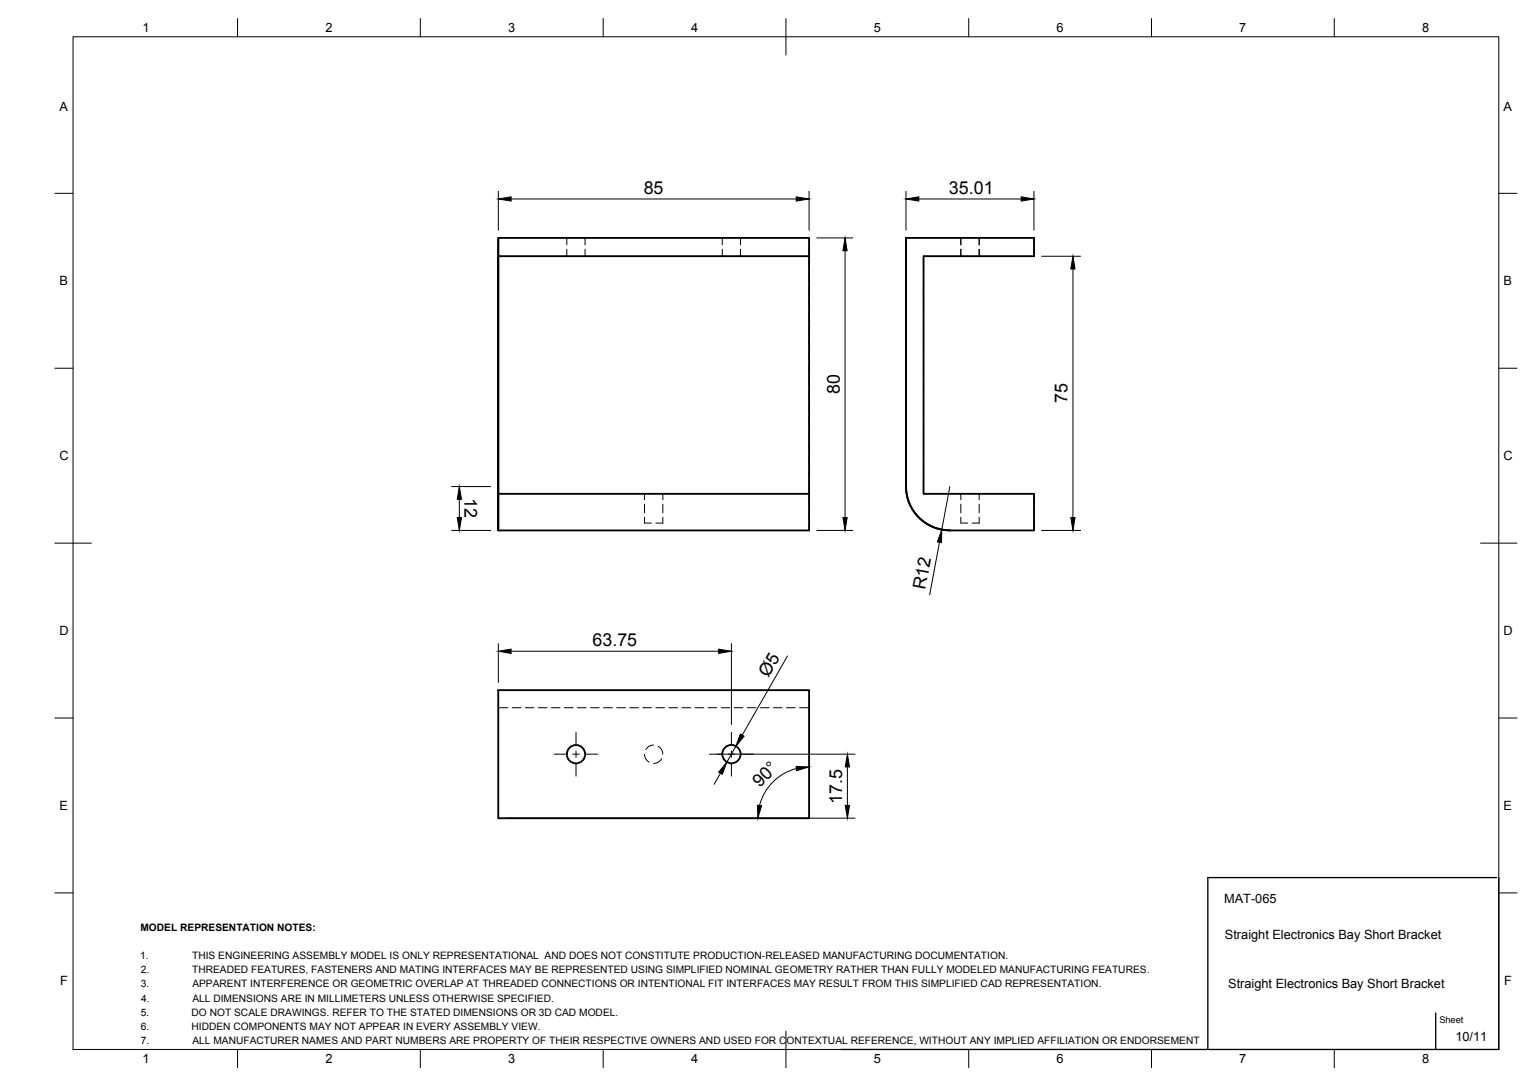
ISO-10303-21;
HEADER;
/* Generated by software containing ST-Developer
 * from STEP Tools, Inc. (www.steptools.com) 
 */

FILE_DESCRIPTION(
/* description */ (
'CAx-IF Rec.Pracs.---Representation and Presentation of Product Manufa
cturing Information (PMI)---4.0---2014-10-13'),
/* implementation_level */ '2;1');

FILE_NAME(
/* name */ 'Straight Electronics Bay Short Bracket.step',
/* time_stamp */ '2026-11-15T23:28:27-08:00',
/* author */ (''),
/* organization */ (''),
/* preprocessor_version */ 'ST-DEVELOPER v20.2',
/* originating_system */ 'Autodesk Translation Framework v15.17.0.0',
/* authorisation */ '');

FILE_SCHEMA (('AUTOMOTIVE_DESIGN { 1 0 10303 214 3 1 1 }'));
ENDSEC;

DATA;
#10=MECHANICAL_DESIGN_GEOMETRIC_PRESENTATION_REPRESENTATION('',(#191),#7756);
#173=SHAPE_REPRESENTATION_RELATIONSHIP('SRR','None',#7821,#182);
#182=ADVANCED_BREP_SHAPE_REPRESENTATION('',(#200),#7749);
#191=STYLED_ITEM('',(#7875),#200);
#200=MANIFOLD_SOLID_BREP('Body1',#4628);
#212=CYLINDRICAL_SURFACE('',#4780,0.0025);
#213=CYLINDRICAL_SURFACE('',#4783,0.0025);
#214=CYLINDRICAL_SURFACE('',#4793,0.012);
#215=CYLINDRICAL_SURFACE('',#4794,0.0025);
#274=CIRCLE('',#4775,0.012);
#275=CIRCLE('',#4778,0.012);
#276=CIRCLE('',#4781,0.0025);
#277=CIRCLE('',#4782,0.0025);
#278=CIRCLE('',#4784,0.0025);
#279=CIRCLE('',#4785,0.0025);
#280=CIRCLE('',#4790,0.0025);
#281=CIRCLE('',#4795,0.0025);
#392=FACE_BOUND('',#731,.T.);
#393=FACE_BOUND('',#732,.T.);
#394=FACE_BOUND('',#734,.T.);
#395=FACE_BOUND('',#735,.T.);
#396=FACE_BOUND('',#738,.T.);
#477=FACE_OUTER_BOUND('',#724,.T.);
#478=FACE_OUTER_BOUND('',#725,.T.);
#479=FACE_OUTER_BOUND('',#726,.T.);
#480=FACE_OUTER_BOUND('',#727,.T.);
#481=FACE_OUTER_BOUND('',#728,.T.);
#482=FACE_OUTER_BOUND('',#729,.T.);
#483=FACE_OUTER_BOUND('',#730,.T.);
#484=FACE_OUTER_BOUND('',#733,.T.);
#485=FACE_OUTER_BOUND('',#736,.T.);
#486=FACE_OUTER_BOUND('',#737,.T.);
#487=FACE_OUTER_BOUND('',#739,.T.);
#488=FACE_OUTER_BOUND('',#740,.T.);
#489=FACE_OUTER_BOUND('',#741,.T.);
#490=FACE_OUTER_BOUND('',#742,.T.);
#491=FACE_OUTER_BOUND('',#743,.T.);
#724=EDGE_LOOP('',(#3119,#3120,#3121,#3122,#3123,#3124,#3125,#3126,#3127));
#725=EDGE_LOOP('',(#3128,#3129,#3130,#3131));
#726=EDGE_LOOP('',(#3132,#3133,#3134,#3135,#3136,#3137,#3138,#3139,#3140));
#727=EDGE_LOOP('',(#3141,#3142,#3143,#3144));
#728=EDGE_LOOP('',(#3145,#3146,#3147,#3148));
#729=EDGE_LOOP('',(#3149,#3150,#3151,#3152));
#730=EDGE_LOOP('',(#3153,#3154,#3155,#3156));
#731=EDGE_LOOP('',(#3157));
#732=EDGE_LOOP('',(#3158));
#733=EDGE_LOOP('',(#3159,#3160,#3161,#3162));
#734=EDGE_LOOP('',(#3163));
#735=EDGE_LOOP('',(#3164));
#736=EDGE_LOOP('',(#3165,#3166,#3167,#3168));
#737=EDGE_LOOP('',(#3169,#3170,#3171,#3172));
#738=EDGE_LOOP('',(#3173));
#739=EDGE_LOOP('',(#3174,#3175,#3176,#3177));
#740=EDGE_LOOP('',(#3178,#3179,#3180,#3181));
#741=EDGE_LOOP('',(#3182,#3183,#3184,#3185));
#742=EDGE_LOOP('',(#3186,#3187,#3188,#3189));
#743=EDGE_LOOP('',(#3190));
#1045=LINE('',#6556,#1538);
#1046=LINE('',#6560,#1539);
#1047=LINE('',#6562,#1540);
#1048=LINE('',#6564,#1541);
#1049=LINE('',#6566,#1542);
#1050=LINE('',#6568,#1543);
#1051=LINE('',#6570,#1544);
#1052=LINE('',#6571,#1545);
#1053=LINE('',#6574,#1546);
#1054=LINE('',#6576,#1547);
#1055=LINE('',#6577,#1548);
#1056=LINE('',#6581,#1549);
#1057=LINE('',#6585,#1550);
#1058=LINE('',#6587,#1551);
#1059=LINE('',#6589,#1552);
#1060=LINE('',#6591,#1553);
#1061=LINE('',#6592,#1554);
#1062=LINE('',#6593,#1555);
#1063=LINE('',#6595,#1556);
#1064=LINE('',#6596,#1557);
#1065=LINE('',#6601,#1558);
#1066=LINE('',#6607,#1559);
#1067=LINE('',#6610,#1560);
#1068=LINE('',#6613,#1561);
#1069=LINE('',#6615,#1562);
#1070=LINE('',#6619,#1563);
#1071=LINE('',#6621,#1564);
#1072=LINE('',#6626,#1565);
#1538=VECTOR('',#5265,1.);
#1539=VECTOR('',#5268,1.);
#1540=VECTOR('',#5269,1.);
#1541=VECTOR('',#5270,1.);
#1542=VECTOR('',#5271,1.);
#1543=VECTOR('',#5272,1.);
#1544=VECTOR('',#5273,1.);
#1545=VECTOR('',#5274,1.);
#1546=VECTOR('',#5277,1.);
#1547=VECTOR('',#5278,1.);
#1548=VECTOR('',#5279,1.);
#1549=VECTOR('',#5282,1.);
#1550=VECTOR('',#5285,1.);
#1551=VECTOR('',#5286,1.);
#1552=VECTOR('',#5287,1.);
#1553=VECTOR('',#5288,1.);
#1554=VECTOR('',#5289,1.);
#1555=VECTOR('',#5290,1.);
#1556=VECTOR('',#5293,1.);
#1557=VECTOR('',#5294,1.);
#1558=VECTOR('',#5299,0.0025);
#1559=VECTOR('',#5306,0.0025);
#1560=VECTOR('',#5311,1.);
#1561=VECTOR('',#5316,1.);
#1562=VECTOR('',#5319,1.);
#1563=VECTOR('',#5324,1.);
#1564=VECTOR('',#5327,1.);
#1565=VECTOR('',#5334,0.0025);
#2020=VERTEX_POINT('',#6554);
#2021=VERTEX_POINT('',#6555);
#2022=VERTEX_POINT('',#6557);
#2023=VERTEX_POINT('',#6559);
#2024=VERTEX_POINT('',#6561);
#2025=VERTEX_POINT('',#6563);
#2026=VERTEX_POINT('',#6565);
#2027=VERTEX_POINT('',#6567);
#2028=VERTEX_POINT('',#6569);
#2029=VERTEX_POINT('',#6573);
#2030=VERTEX_POINT('',#6575);
#2031=VERTEX_POINT('',#6579);
#2032=VERTEX_POINT('',#6580);
#2033=VERTEX_POINT('',#6582);
#2034=VERTEX_POINT('',#6584);
#2035=VERTEX_POINT('',#6586);
#2036=VERTEX_POINT('',#6588);
#2037=VERTEX_POINT('',#6590);
#2038=VERTEX_POINT('',#6598);
#2039=VERTEX_POINT('',#6600);
#2040=VERTEX_POINT('',#6604);
#2041=VERTEX_POINT('',#6606);
#2042=VERTEX_POINT('',#6616);
#2043=VERTEX_POINT('',#6624);
#2443=EDGE_CURVE('',#2020,#2021,#1045,.T.);
#2444=EDGE_CURVE('',#2021,#2022,#274,.T.);
#2445=EDGE_CURVE('',#2022,#2023,#1046,.T.);
#2446=EDGE_CURVE('',#2024,#2023,#1047,.T.);
#2447=EDGE_CURVE('',#2025,#2024,#1048,.T.);
#2448=EDGE_CURVE('',#2025,#2026,#1049,.T.);
#2449=EDGE_CURVE('',#2027,#2026,#1050,.T.);
#2450=EDGE_CURVE('',#2028,#2027,#1051,.T.);
#2451=EDGE_CURVE('',#2020,#2028,#1052,.T.);
#2452=EDGE_CURVE('',#2024,#2029,#1053,.T.);
#2453=EDGE_CURVE('',#2030,#2029,#1054,.T.);
#2454=EDGE_CURVE('',#2025,#2030,#1055,.T.);
#2455=EDGE_CURVE('',#2031,#2032,#1056,.T.);
#2456=EDGE_CURVE('',#2031,#2033,#275,.F.);
#2457=EDGE_CURVE('',#2034,#2033,#1057,.T.);
#2458=EDGE_CURVE('',#2034,#2035,#1058,.T.);
#2459=EDGE_CURVE('',#2035,#2036,#1059,.T.);
#2460=EDGE_CURVE('',#2036,#2037,#1060,.T.);
#2461=EDGE_CURVE('',#2030,#2037,#1061,.T.);
#2462=EDGE_CURVE('',#2029,#2032,#1062,.T.);
#2463=EDGE_CURVE('',#2022,#2031,#1063,.T.);
#2464=EDGE_CURVE('',#2023,#2032,#1064,.T.);
#2465=EDGE_CURVE('',#2038,#2038,#276,.T.);
#2466=EDGE_CURVE('',#2038,#2039,#1065,.T.);
#2467=EDGE_CURVE('',#2039,#2039,#277,.T.);
#2468=EDGE_CURVE('',#2040,#2040,#278,.T.);
#2469=EDGE_CURVE('',#2040,#2041,#1066,.T.);
#2470=EDGE_CURVE('',#2041,#2041,#279,.T.);
#2471=EDGE_CURVE('',#2026,#2037,#1067,.T.);
#2472=EDGE_CURVE('',#2027,#2036,#1068,.T.);
#2473=EDGE_CURVE('',#2028,#2035,#1069,.T.);
#2474=EDGE_CURVE('',#2042,#2042,#280,.T.);
#2475=EDGE_CURVE('',#2020,#2034,#1070,.T.);
#2476=EDGE_CURVE('',#2033,#2021,#1071,.F.);
#2477=EDGE_CURVE('',#2043,#2043,#281,.T.);
#2478=EDGE_CURVE('',#2043,#2042,#1072,.T.);
#3119=ORIENTED_EDGE('',*,*,#2443,.T.);
#3120=ORIENTED_EDGE('',*,*,#2444,.T.);
#3121=ORIENTED_EDGE('',*,*,#2445,.T.);
#3122=ORIENTED_EDGE('',*,*,#2446,.F.);
#3123=ORIENTED_EDGE('',*,*,#2447,.F.);
#3124=ORIENTED_EDGE('',*,*,#2448,.T.);
#3125=ORIENTED_EDGE('',*,*,#2449,.F.);
#3126=ORIENTED_EDGE('',*,*,#2450,.F.);
#3127=ORIENTED_EDGE('',*,*,#2451,.F.);
#3128=ORIENTED_EDGE('',*,*,#2452,.T.);
#3129=ORIENTED_EDGE('',*,*,#2453,.F.);
#3130=ORIENTED_EDGE('',*,*,#2454,.F.);
#3131=ORIENTED_EDGE('',*,*,#2447,.T.);
#3132=ORIENTED_EDGE('',*,*,#2455,.F.);
#3133=ORIENTED_EDGE('',*,*,#2456,.T.);
#3134=ORIENTED_EDGE('',*,*,#2457,.F.);
#3135=ORIENTED_EDGE('',*,*,#2458,.T.);
#3136=ORIENTED_EDGE('',*,*,#2459,.T.);
#3137=ORIENTED_EDGE('',*,*,#2460,.T.);
#3138=ORIENTED_EDGE('',*,*,#2461,.F.);
#3139=ORIENTED_EDGE('',*,*,#2453,.T.);
#3140=ORIENTED_EDGE('',*,*,#2462,.T.);
#3141=ORIENTED_EDGE('',*,*,#2445,.F.);
#3142=ORIENTED_EDGE('',*,*,#2463,.T.);
#3143=ORIENTED_EDGE('',*,*,#2455,.T.);
#3144=ORIENTED_EDGE('',*,*,#2464,.F.);
#3145=ORIENTED_EDGE('',*,*,#2465,.F.);
#3146=ORIENTED_EDGE('',*,*,#2466,.T.);
#3147=ORIENTED_EDGE('',*,*,#2467,.T.);
#3148=ORIENTED_EDGE('',*,*,#2466,.F.);
#3149=ORIENTED_EDGE('',*,*,#2468,.F.);
#3150=ORIENTED_EDGE('',*,*,#2469,.T.);
#3151=ORIENTED_EDGE('',*,*,#2470,.T.);
#3152=ORIENTED_EDGE('',*,*,#2469,.F.);
#3153=ORIENTED_EDGE('',*,*,#2471,.F.);
#3154=ORIENTED_EDGE('',*,*,#2448,.F.);
#3155=ORIENTED_EDGE('',*,*,#2454,.T.);
#3156=ORIENTED_EDGE('',*,*,#2461,.T.);
#3157=ORIENTED_EDGE('',*,*,#2465,.T.);
#3158=ORIENTED_EDGE('',*,*,#2468,.T.);
#3159=ORIENTED_EDGE('',*,*,#2446,.T.);
#3160=ORIENTED_EDGE('',*,*,#2464,.T.);
#3161=ORIENTED_EDGE('',*,*,#2462,.F.);
#3162=ORIENTED_EDGE('',*,*,#2452,.F.);
#3163=ORIENTED_EDGE('',*,*,#2470,.F.);
#3164=ORIENTED_EDGE('',*,*,#2467,.F.);
#3165=ORIENTED_EDGE('',*,*,#2471,.T.);
#3166=ORIENTED_EDGE('',*,*,#2460,.F.);
#3167=ORIENTED_EDGE('',*,*,#2472,.F.);
#3168=ORIENTED_EDGE('',*,*,#2449,.T.);
#3169=ORIENTED_EDGE('',*,*,#2450,.T.);
#3170=ORIENTED_EDGE('',*,*,#2472,.T.);
#3171=ORIENTED_EDGE('',*,*,#2459,.F.);
#3172=ORIENTED_EDGE('',*,*,#2473,.F.);
#3173=ORIENTED_EDGE('',*,*,#2474,.F.);
#3174=ORIENTED_EDGE('',*,*,#2473,.T.);
#3175=ORIENTED_EDGE('',*,*,#2458,.F.);
#3176=ORIENTED_EDGE('',*,*,#2475,.F.);
#3177=ORIENTED_EDGE('',*,*,#2451,.T.);
#3178=ORIENTED_EDGE('',*,*,#2457,.T.);
#3179=ORIENTED_EDGE('',*,*,#2476,.T.);
#3180=ORIENTED_EDGE('',*,*,#2443,.F.);
#3181=ORIENTED_EDGE('',*,*,#2475,.T.);
#3182=ORIENTED_EDGE('',*,*,#2444,.F.);
#3183=ORIENTED_EDGE('',*,*,#2476,.F.);
#3184=ORIENTED_EDGE('',*,*,#2456,.F.);
#3185=ORIENTED_EDGE('',*,*,#2463,.F.);
#3186=ORIENTED_EDGE('',*,*,#2477,.F.);
#3187=ORIENTED_EDGE('',*,*,#2478,.T.);
#3188=ORIENTED_EDGE('',*,*,#2474,.T.);
#3189=ORIENTED_EDGE('',*,*,#2478,.F.);
#3190=ORIENTED_EDGE('',*,*,#2477,.T.);
#4239=PLANE('',#4774);
#4240=PLANE('',#4776);
#4241=PLANE('',#4777);
#4242=PLANE('',#4779);
#4243=PLANE('',#4786);
#4244=PLANE('',#4787);
#4245=PLANE('',#4788);
#4246=PLANE('',#4789);
#4247=PLANE('',#4791);
#4248=PLANE('',#4792);
#4249=PLANE('',#4796);
#4418=ADVANCED_FACE('',(#477),#4239,.T.);
#4419=ADVANCED_FACE('',(#478),#4240,.F.);
#4420=ADVANCED_FACE('',(#479),#4241,.F.);
#4421=ADVANCED_FACE('',(#480),#4242,.T.);
#4422=ADVANCED_FACE('',(#481),#212,.F.);
#4423=ADVANCED_FACE('',(#482),#213,.F.);
#4424=ADVANCED_FACE('',(#483,#392,#393),#4243,.T.);
#4425=ADVANCED_FACE('',(#484,#394,#395),#4244,.F.);
#4426=ADVANCED_FACE('',(#485),#4245,.F.);
#4427=ADVANCED_FACE('',(#486,#396),#4246,.F.);
#4428=ADVANCED_FACE('',(#487),#4247,.F.);
#4429=ADVANCED_FACE('',(#488),#4248,.T.);
#4430=ADVANCED_FACE('',(#489),#214,.T.);
#4431=ADVANCED_FACE('',(#490),#215,.F.);
#4432=ADVANCED_FACE('',(#491),#4249,.T.);
#4628=CLOSED_SHELL('',(#4418,#4419,#4420,#4421,#4422,#4423,#4424,#4425,
#4426,#4427,#4428,#4429,#4430,#4431,#4432));
#4773=AXIS2_PLACEMENT_3D('',#6552,#5261,#5262);
#4774=AXIS2_PLACEMENT_3D('',#6553,#5263,#5264);
#4775=AXIS2_PLACEMENT_3D('',#6558,#5266,#5267);
#4776=AXIS2_PLACEMENT_3D('',#6572,#5275,#5276);
#4777=AXIS2_PLACEMENT_3D('',#6578,#5280,#5281);
#4778=AXIS2_PLACEMENT_3D('',#6583,#5283,#5284);
#4779=AXIS2_PLACEMENT_3D('',#6594,#5291,#5292);
#4780=AXIS2_PLACEMENT_3D('',#6597,#5295,#5296);
#4781=AXIS2_PLACEMENT_3D('',#6599,#5297,#5298);
#4782=AXIS2_PLACEMENT_3D('',#6602,#5300,#5301);
#4783=AXIS2_PLACEMENT_3D('',#6603,#5302,#5303);
#4784=AXIS2_PLACEMENT_3D('',#6605,#5304,#5305);
#4785=AXIS2_PLACEMENT_3D('',#6608,#5307,#5308);
#4786=AXIS2_PLACEMENT_3D('',#6609,#5309,#5310);
#4787=AXIS2_PLACEMENT_3D('',#6611,#5312,#5313);
#4788=AXIS2_PLACEMENT_3D('',#6612,#5314,#5315);
#4789=AXIS2_PLACEMENT_3D('',#6614,#5317,#5318);
#4790=AXIS2_PLACEMENT_3D('',#6617,#5320,#5321);
#4791=AXIS2_PLACEMENT_3D('',#6618,#5322,#5323);
#4792=AXIS2_PLACEMENT_3D('',#6620,#5325,#5326);
#4793=AXIS2_PLACEMENT_3D('',#6622,#5328,#5329);
#4794=AXIS2_PLACEMENT_3D('',#6623,#5330,#5331);
#4795=AXIS2_PLACEMENT_3D('',#6625,#5332,#5333);
#4796=AXIS2_PLACEMENT_3D('',#6627,#5335,#5336);
#5261=DIRECTION('axis',(0.,0.,1.));
#5262=DIRECTION('refdir',(1.,0.,0.));
#5263=DIRECTION('center_axis',(-1.,0.,0.));
#5264=DIRECTION('ref_axis',(0.,0.,1.));
#5265=DIRECTION('',(0.,-1.,0.));
#5266=DIRECTION('center_axis',(-1.,0.,0.));
#5267=DIRECTION('ref_axis',(0.,0.,1.));
#5268=DIRECTION('',(0.,0.,1.));
#5269=DIRECTION('',(0.,-1.,0.));
#5270=DIRECTION('',(0.,0.,1.));
#5271=DIRECTION('',(0.,-1.,0.));
#5272=DIRECTION('',(0.,0.,1.));
#5273=DIRECTION('',(0.,-1.,0.));
#5274=DIRECTION('',(0.,0.,1.));
#5275=DIRECTION('center_axis',(2.04085114820801E-16,-1.,0.));
#5276=DIRECTION('ref_axis',(1.,2.04085114820801E-16,0.));
#5277=DIRECTION('',(1.,2.04085114820801E-16,0.));
#5278=DIRECTION('',(0.,0.,1.));
#5279=DIRECTION('',(1.,2.04085114820801E-16,0.));
#5280=DIRECTION('center_axis',(-1.,0.,0.));
#5281=DIRECTION('ref_axis',(0.,0.,1.));
#5282=DIRECTION('',(0.,0.,1.));
#5283=DIRECTION('center_axis',(-1.,0.,0.));
#5284=DIRECTION('ref_axis',(0.,0.,1.));
#5285=DIRECTION('',(0.,-1.,0.));
#5286=DIRECTION('',(0.,0.,1.));
#5287=DIRECTION('',(0.,-1.,0.));
#5288=DIRECTION('',(0.,0.,1.));
#5289=DIRECTION('',(0.,-1.,0.));
#5290=DIRECTION('',(0.,-1.,0.));
#5291=DIRECTION('center_axis',(1.6326809185664E-16,-1.,0.));
#5292=DIRECTION('ref_axis',(1.,1.6326809185664E-16,0.));
#5293=DIRECTION('',(1.,1.6326809185664E-16,0.));
#5294=DIRECTION('',(1.,1.6326809185664E-16,0.));
#5295=DIRECTION('center_axis',(0.,0.,1.));
#5296=DIRECTION('ref_axis',(1.,0.,0.));
#5297=DIRECTION('center_axis',(0.,0.,1.));
#5298=DIRECTION('ref_axis',(1.,0.,0.));
#5299=DIRECTION('',(0.,0.,1.));
#5300=DIRECTION('center_axis',(0.,0.,1.));
#5301=DIRECTION('ref_axis',(1.,0.,0.));
#5302=DIRECTION('center_axis',(0.,0.,1.));
#5303=DIRECTION('ref_axis',(1.,0.,0.));
#5304=DIRECTION('center_axis',(0.,0.,1.));
#5305=DIRECTION('ref_axis',(1.,0.,0.));
#5306=DIRECTION('',(0.,0.,1.));
#5307=DIRECTION('center_axis',(0.,0.,1.));
#5308=DIRECTION('ref_axis',(1.,0.,0.));
#5309=DIRECTION('center_axis',(0.,0.,-1.));
#5310=DIRECTION('ref_axis',(1.,0.,0.));
#5311=DIRECTION('',(1.,0.,0.));
#5312=DIRECTION('center_axis',(0.,0.,-1.));
#5313=DIRECTION('ref_axis',(1.,0.,0.));
#5314=DIRECTION('center_axis',(0.,-1.,0.));
#5315=DIRECTION('ref_axis',(0.,0.,-1.));
#5316=DIRECTION('',(1.,0.,0.));
#5317=DIRECTION('center_axis',(0.,0.,-1.));
#5318=DIRECTION('ref_axis',(1.,0.,0.));
#5319=DIRECTION('',(1.,0.,0.));
#5320=DIRECTION('center_axis',(0.,0.,1.));
#5321=DIRECTION('ref_axis',(1.,0.,0.));
#5322=DIRECTION('center_axis',(0.,-1.,0.));
#5323=DIRECTION('ref_axis',(0.,0.,-1.));
#5324=DIRECTION('',(1.,0.,0.));
#5325=DIRECTION('center_axis',(0.,0.,-1.));
#5326=DIRECTION('ref_axis',(1.,0.,0.));
#5327=DIRECTION('',(1.,1.6326809185664E-16,0.));
#5328=DIRECTION('center_axis',(1.,1.6326809185664E-16,0.));
#5329=DIRECTION('ref_axis',(-1.6326809185664E-16,1.,0.));
#5330=DIRECTION('center_axis',(0.,0.,1.));
#5331=DIRECTION('ref_axis',(1.,0.,0.));
#5332=DIRECTION('center_axis',(0.,0.,1.));
#5333=DIRECTION('ref_axis',(1.,0.,0.));
#5334=DIRECTION('',(0.,0.,1.));
#5335=DIRECTION('center_axis',(0.,0.,1.));
#5336=DIRECTION('ref_axis',(1.,0.,0.));
#6552=CARTESIAN_POINT('',(0.,0.,0.));
#6553=CARTESIAN_POINT('Origin',(-0.0425,-3.46944695195361E-18,-0.005));
#6554=CARTESIAN_POINT('',(-0.0425,0.0175,-0.08));
#6555=CARTESIAN_POINT('',(-0.0425,-0.0055,-0.08));
#6556=CARTESIAN_POINT('',(-0.0425,-3.46944695195361E-18,-0.08));
#6557=CARTESIAN_POINT('',(-0.0425,-0.0175,-0.068));
#6558=CARTESIAN_POINT('Origin',(-0.0425,-0.0055,-0.068));
#6559=CARTESIAN_POINT('',(-0.0425,-0.0175,0.));
#6560=CARTESIAN_POINT('',(-0.0425,-0.0175,-0.005));
#6561=CARTESIAN_POINT('',(-0.0425,0.0175,0.));
#6562=CARTESIAN_POINT('',(-0.0425,-3.46944695195361E-18,0.));
#6563=CARTESIAN_POINT('',(-0.0425,0.0175,-0.005));
#6564=CARTESIAN_POINT('',(-0.0425,0.0175,-0.005));
#6565=CARTESIAN_POINT('',(-0.0425,-0.0127,-0.005));
#6566=CARTESIAN_POINT('',(-0.0425,-3.46944695195361E-18,-0.005));
#6567=CARTESIAN_POINT('',(-0.0425,-0.0127,-0.07));
#6568=CARTESIAN_POINT('',(-0.0425,-0.0127,-0.07));
#6569=CARTESIAN_POINT('',(-0.0425,0.0175,-0.07));
#6570=CARTESIAN_POINT('',(-0.0425,-3.46944695195361E-18,-0.07));
#6571=CARTESIAN_POINT('',(-0.0425,0.0175,-0.08));
#6572=CARTESIAN_POINT('Origin',(0.,0.0175,-0.005));
#6573=CARTESIAN_POINT('',(0.0425,0.0175,0.));
#6574=CARTESIAN_POINT('',(0.,0.0175,0.));
#6575=CARTESIAN_POINT('',(0.0425,0.0175,-0.005));
#6576=CARTESIAN_POINT('',(0.0425,0.0175,-0.005));
#6577=CARTESIAN_POINT('',(0.,0.0175,-0.005));
#6578=CARTESIAN_POINT('Origin',(0.0425,1.04083408558608E-17,-0.005));
#6579=CARTESIAN_POINT('',(0.0425,-0.0175,-0.068));
#6580=CARTESIAN_POINT('',(0.0425,-0.0175,0.));
#6581=CARTESIAN_POINT('',(0.0425,-0.0175,-0.005));
#6582=CARTESIAN_POINT('',(0.0425,-0.0055,-0.08));
#6583=CARTESIAN_POINT('Origin',(0.0425,-0.0055,-0.068));
#6584=CARTESIAN_POINT('',(0.0425,0.0175,-0.08));
#6585=CARTESIAN_POINT('',(0.0425,1.04083408558608E-17,-0.08));
#6586=CARTESIAN_POINT('',(0.0425,0.0175,-0.07));
#6587=CARTESIAN_POINT('',(0.0425,0.0175,-0.08));
#6588=CARTESIAN_POINT('',(0.0425,-0.0127,-0.07));
#6589=CARTESIAN_POINT('',(0.0425,1.04083408558608E-17,-0.07));
#6590=CARTESIAN_POINT('',(0.0425,-0.0127,-0.005));
#6591=CARTESIAN_POINT('',(0.0425,-0.0127,-0.07));
#6592=CARTESIAN_POINT('',(0.0425,1.04083408558608E-17,-0.005));
#6593=CARTESIAN_POINT('',(0.0425,1.04083408558608E-17,0.));
#6594=CARTESIAN_POINT('Origin',(0.,-0.0175,-0.005));
#6595=CARTESIAN_POINT('',(0.,-0.0175,-0.068));
#6596=CARTESIAN_POINT('',(0.,-0.0175,0.));
#6597=CARTESIAN_POINT('Origin',(0.02125,4.59242549680257E-19,-0.005));
#6598=CARTESIAN_POINT('',(0.01875,1.53080849893419E-19,-0.005));
#6599=CARTESIAN_POINT('Origin',(0.02125,4.59242549680257E-19,-0.005));
#6600=CARTESIAN_POINT('',(0.01875,1.53080849893419E-19,0.));
#6601=CARTESIAN_POINT('',(0.01875,1.53080849893419E-19,-0.005));
#6602=CARTESIAN_POINT('Origin',(0.02125,4.59242549680257E-19,0.));
#6603=CARTESIAN_POINT('Origin',(-0.02125,1.53080849893419E-19,-0.005));
#6604=CARTESIAN_POINT('',(-0.02375,-1.53080849893419E-19,-0.005));
#6605=CARTESIAN_POINT('Origin',(-0.02125,1.53080849893419E-19,-0.005));
#6606=CARTESIAN_POINT('',(-0.02375,-1.53080849893419E-19,0.));
#6607=CARTESIAN_POINT('',(-0.02375,-1.53080849893419E-19,-0.005));
#6608=CARTESIAN_POINT('Origin',(-0.02125,1.53080849893419E-19,0.));
#6609=CARTESIAN_POINT('Origin',(0.,3.46944695195361E-18,-0.005));
#6610=CARTESIAN_POINT('',(0.,-0.0127,-0.005));
#6611=CARTESIAN_POINT('Origin',(0.,3.46944695195361E-18,0.));
#6612=CARTESIAN_POINT('Origin',(0.,-0.0127,-0.07));
#6613=CARTESIAN_POINT('',(0.,-0.0127,-0.07));
#6614=CARTESIAN_POINT('Origin',(6.93889390390723E-18,0.,-0.07));
#6615=CARTESIAN_POINT('',(6.93889390390723E-18,0.0175,-0.07));
#6616=CARTESIAN_POINT('',(-0.0025,-1.53080849893419E-19,-0.07));
#6617=CARTESIAN_POINT('Origin',(0.,1.53080849893419E-19,-0.07));
#6618=CARTESIAN_POINT('Origin',(6.93889390390723E-18,0.0175,-0.08));
#6619=CARTESIAN_POINT('',(6.93889390390723E-18,0.0175,-0.08));
#6620=CARTESIAN_POINT('Origin',(6.93889390390723E-18,0.,-0.08));
#6621=CARTESIAN_POINT('',(7.83686840911875E-18,-0.0055,-0.08));
#6622=CARTESIAN_POINT('Origin',(-1.95921710227969E-18,-0.0055,-0.068));
#6623=CARTESIAN_POINT('Origin',(0.,1.53080849893419E-19,-0.078));
#6624=CARTESIAN_POINT('',(-0.0025,-1.53080849893419E-19,-0.078));
#6625=CARTESIAN_POINT('Origin',(0.,1.53080849893419E-19,-0.078));
#6626=CARTESIAN_POINT('',(-0.0025,-1.53080849893419E-19,-0.078));
#6627=CARTESIAN_POINT('Origin',(6.93889390390723E-18,0.0024,-0.078));
#7738=UNCERTAINTY_MEASURE_WITH_UNIT(LENGTH_MEASURE(1.E-5),#7757,
'DISTANCE_ACCURACY_VALUE',
'Maximum model space distance between geometric entities at asserted c
onnectivities');
#7745=UNCERTAINTY_MEASURE_WITH_UNIT(LENGTH_MEASURE(1.E-5),#7757,
'DISTANCE_ACCURACY_VALUE',
'Maximum model space distance between geometric entities at asserted c
onnectivities');
#7749=(
GEOMETRIC_REPRESENTATION_CONTEXT(3)
GLOBAL_UNCERTAINTY_ASSIGNED_CONTEXT((#7738))
GLOBAL_UNIT_ASSIGNED_CONTEXT((#7757,#7758,#7759))
REPRESENTATION_CONTEXT('','3D')
);
#7756=(
GEOMETRIC_REPRESENTATION_CONTEXT(3)
GLOBAL_UNCERTAINTY_ASSIGNED_CONTEXT((#7745))
GLOBAL_UNIT_ASSIGNED_CONTEXT((#7757,#7758,#7759))
REPRESENTATION_CONTEXT('','3D')
);
#7757=(
LENGTH_UNIT()
NAMED_UNIT(*)
SI_UNIT($,.METRE.)
);
#7758=(
NAMED_UNIT(*)
PLANE_ANGLE_UNIT()
SI_UNIT($,.RADIAN.)
);
#7759=(
NAMED_UNIT(*)
SI_UNIT($,.STERADIAN.)
SOLID_ANGLE_UNIT()
);
#7763=SHAPE_DEFINITION_REPRESENTATION(#7773,#7821);
#7773=PRODUCT_DEFINITION_SHAPE('',$,#7832);
#7821=SHAPE_REPRESENTATION('',(#4773),#7749);
#7828=PRODUCT_DEFINITION_CONTEXT('part definition',#7860,'design');
#7832=PRODUCT_DEFINITION('Straight Electronics Bay Short Bracket',
'Straight Electronics Bay Short Bracket',#7842,#7828);
#7842=PRODUCT_DEFINITION_FORMATION('',$,#7865);
#7860=APPLICATION_CONTEXT(
'Core Data for Automotive Mechanical Design Process');
#7861=PRODUCT_CONTEXT('part definition',#7860,'mechanical');
#7865=PRODUCT('Straight Electronics Bay Short Bracket',
'Straight Electronics Bay Short Bracket',
'LEGAL AND USAGE DISCLAIMER: this Data/Model is provided \X2\201C\X0\A
S IS\X2\201D\X0\ for informational and representational only. It is a 
geometric approximation and is NOT engineered, certified, or guarantee
d for dimensional accuracy, exact tolerances, or production-level prec
ision. Vendor disclaims all implied warranties including fitness for a
 particular purpose. DO NOT USE FOR DIRECT PHYSICAL MANUFACTURING, AUT
OMATED PRODUCTION, OR SAFETY-CRITICAL SYSTEMS without independent engi
neering verification and resolution of any design discrepancies.',(#7861));
#7875=PRESENTATION_STYLE_ASSIGNMENT((#7882));
#7882=SURFACE_STYLE_USAGE(.BOTH.,#7889);
#7889=SURFACE_SIDE_STYLE('',(#7896));
#7896=SURFACE_STYLE_FILL_AREA(#7903);
#7903=FILL_AREA_STYLE('Opaque(25,25,25)',(#7910));
#7910=FILL_AREA_STYLE_COLOUR('Opaque(25,25,25)',#7917);
#7917=COLOUR_RGB('Opaque(25,25,25)',0.0980392156862745,0.0980392156862745,
0.0980392156862745);
ENDSEC;
END-ISO-10303-21;
